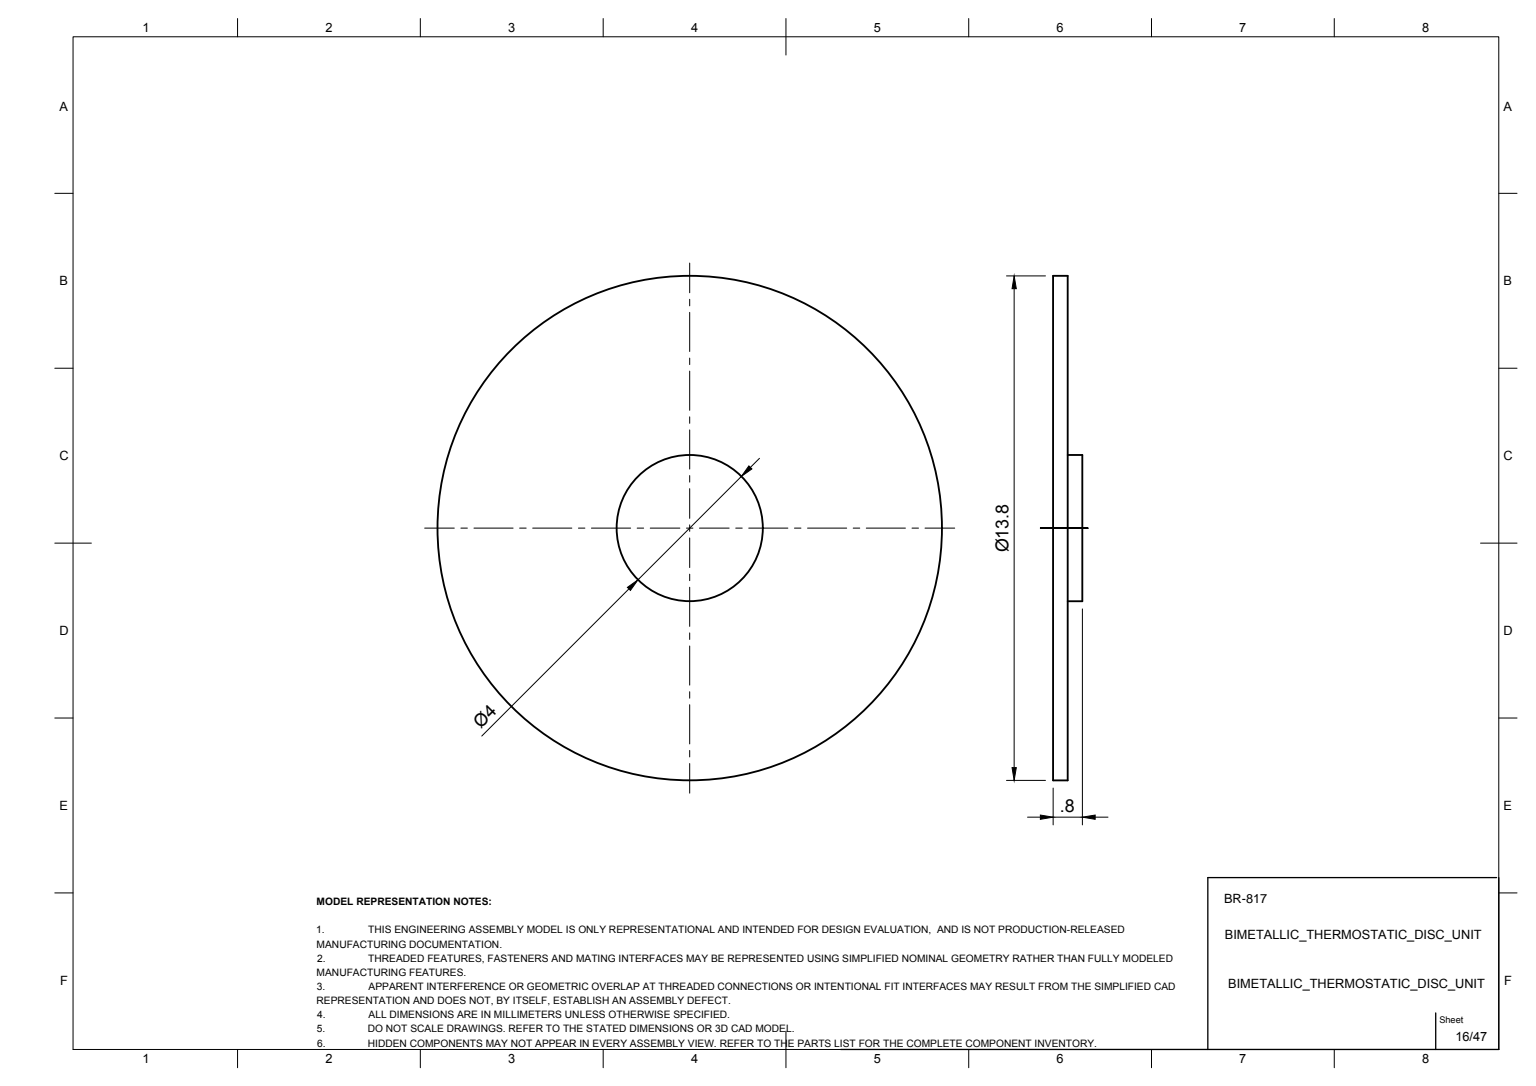
ISO-10303-21;
HEADER;
FILE_DESCRIPTION((''),'2;1');
FILE_NAME('BIMETALLIC_THERMOSTATIC_DISC_UNIT.step','2026-10-01T22:07:29-07:00',(''),(''),'','','');
FILE_SCHEMA (('AUTOMOTIVE_DESIGN { 1 0 10303 214 3 1 1 }'));
ENDSEC;
DATA;
#10=MECHANICAL_DESIGN_GEOMETRIC_PRESENTATION_REPRESENTATION('',(#550),#15484);
#480=SHAPE_REPRESENTATION_RELATIONSHIP('SRR','None',#15629,#515) ;
#515=ADVANCED_BREP_SHAPE_REPRESENTATION('',(#592),#15453) ;
#550=STYLED_ITEM('',(#15835),#592) ;
#592=MANIFOLD_SOLID_BREP('BIMETALLIC_THERMOSTATIC_DISC_UNIT',#8259) ;
#660=CYLINDRICAL_SURFACE('',#8884,0.2) ;
#661=CYLINDRICAL_SURFACE('',#8888,0.69) ;
#852=FACE_BOUND('',#2027,.T.) ;
#954=CIRCLE('',#8885,0.2) ;
#955=CIRCLE('',#8886,0.2) ;
#956=CIRCLE('',#8889,0.69) ;
#957=CIRCLE('',#8890,0.69) ;
#1480=FACE_OUTER_BOUND('',#2022,.T.) ;
#1481=FACE_OUTER_BOUND('',#2023,.T.) ;
#1482=FACE_OUTER_BOUND('',#2024,.T.) ;
#1483=FACE_OUTER_BOUND('',#2025,.T.) ;
#1484=FACE_OUTER_BOUND('',#2026,.T.) ;
#2022=EDGE_LOOP('',(#5761,#5762,#5763,#5764)) ;
#2023=EDGE_LOOP('',(#5765)) ;
#2024=EDGE_LOOP('',(#5766,#5767,#5768,#5769)) ;
#2025=EDGE_LOOP('',(#5770)) ;
#2026=EDGE_LOOP('',(#5771)) ;
#2027=EDGE_LOOP('',(#5772)) ;
#2615=LINE('',#13429,#3089) ;
#2616=LINE('',#13436,#3090) ;
#3089=VECTOR('',#10508,0.2) ;
#3090=VECTOR('',#10517,0.69) ;
#3551=VERTEX_POINT('',#13426) ;
#3552=VERTEX_POINT('',#13428) ;
#3553=VERTEX_POINT('',#13433) ;
#3554=VERTEX_POINT('',#13435) ;
#4385=EDGE_CURVE('',#3551,#3551,#954,.T.) ;
#4386=EDGE_CURVE('',#3551,#3552,#2615,.T.) ;
#4387=EDGE_CURVE('',#3552,#3552,#955,.T.) ;
#4388=EDGE_CURVE('',#3553,#3553,#956,.T.) ;
#4389=EDGE_CURVE('',#3553,#3554,#2616,.T.) ;
#4390=EDGE_CURVE('',#3554,#3554,#957,.T.) ;
#5761=ORIENTED_EDGE('',*,*,#4385,.F.) ;
#5762=ORIENTED_EDGE('',*,*,#4386,.T.) ;
#5763=ORIENTED_EDGE('',*,*,#4387,.F.) ;
#5764=ORIENTED_EDGE('',*,*,#4386,.F.) ;
#5765=ORIENTED_EDGE('',*,*,#4385,.T.) ;
#5766=ORIENTED_EDGE('',*,*,#4388,.F.) ;
#5767=ORIENTED_EDGE('',*,*,#4389,.T.) ;
#5768=ORIENTED_EDGE('',*,*,#4390,.F.) ;
#5769=ORIENTED_EDGE('',*,*,#4389,.F.) ;
#5770=ORIENTED_EDGE('',*,*,#4390,.T.) ;
#5771=ORIENTED_EDGE('',*,*,#4388,.T.) ;
#5772=ORIENTED_EDGE('',*,*,#4387,.T.) ;
#7617=PLANE('',#8887) ;
#7618=PLANE('',#8891) ;
#7619=PLANE('',#8892) ;
#7867=ADVANCED_FACE('',(#1480),#660,.T.) ;
#7868=ADVANCED_FACE('',(#1481),#7617,.T.) ;
#7869=ADVANCED_FACE('',(#1482),#661,.T.) ;
#7870=ADVANCED_FACE('',(#1483),#7618,.T.) ;
#7871=ADVANCED_FACE('',(#1484,#852),#7619,.T.) ;
#8259=CLOSED_SHELL('',(#7867,#7868,#7869,#7870,#7871)) ;
#8883=AXIS2_PLACEMENT_3D('',#13424,#10502,#10503) ;
#8884=AXIS2_PLACEMENT_3D('',#13425,#10504,#10505) ;
#8885=AXIS2_PLACEMENT_3D('',#13427,#10506,#10507) ;
#8886=AXIS2_PLACEMENT_3D('',#13430,#10509,#10510) ;
#8887=AXIS2_PLACEMENT_3D('',#13431,#10511,#10512) ;
#8888=AXIS2_PLACEMENT_3D('',#13432,#10513,#10514) ;
#8889=AXIS2_PLACEMENT_3D('',#13434,#10515,#10516) ;
#8890=AXIS2_PLACEMENT_3D('',#13437,#10518,#10519) ;
#8891=AXIS2_PLACEMENT_3D('',#13438,#10520,#10521) ;
#8892=AXIS2_PLACEMENT_3D('',#13439,#10522,#10523) ;
#10502=DIRECTION('axis',(0.,0.,1.)) ;
#10503=DIRECTION('refdir',(1.,0.,0.)) ;
#10504=DIRECTION('center_axis',(0.,0.,1.)) ;
#10505=DIRECTION('ref_axis',(1.,0.,0.)) ;
#10506=DIRECTION('center_axis',(0.,0.,1.)) ;
#10507=DIRECTION('ref_axis',(1.,0.,0.)) ;
#10508=DIRECTION('',(0.,0.,-1.)) ;
#10509=DIRECTION('center_axis',(0.,0.,-1.)) ;
#10510=DIRECTION('ref_axis',(1.,0.,0.)) ;
#10511=DIRECTION('center_axis',(0.,0.,1.)) ;
#10512=DIRECTION('ref_axis',(1.,0.,0.)) ;
#10513=DIRECTION('center_axis',(0.,0.,1.)) ;
#10514=DIRECTION('ref_axis',(1.,0.,0.)) ;
#10515=DIRECTION('center_axis',(0.,0.,1.)) ;
#10516=DIRECTION('ref_axis',(1.,0.,0.)) ;
#10517=DIRECTION('',(0.,0.,-1.)) ;
#10518=DIRECTION('center_axis',(0.,0.,-1.)) ;
#10519=DIRECTION('ref_axis',(1.,0.,0.)) ;
#10520=DIRECTION('center_axis',(0.,0.,-1.)) ;
#10521=DIRECTION('ref_axis',(-1.,0.,0.)) ;
#10522=DIRECTION('center_axis',(0.,0.,1.)) ;
#10523=DIRECTION('ref_axis',(1.,0.,0.)) ;
#13424=CARTESIAN_POINT('',(0.,0.,0.)) ;
#13425=CARTESIAN_POINT('Origin',(2.,0.8,1.11)) ;
#13426=CARTESIAN_POINT('',(1.8,0.8,1.13)) ;
#13427=CARTESIAN_POINT('Origin',(2.,0.8,1.13)) ;
#13428=CARTESIAN_POINT('',(1.8,0.8,1.09)) ;
#13429=CARTESIAN_POINT('',(1.8,0.8,1.11)) ;
#13430=CARTESIAN_POINT('Origin',(2.,0.8,1.09)) ;
#13431=CARTESIAN_POINT('Origin',(2.,0.8,1.13)) ;
#13432=CARTESIAN_POINT('Origin',(2.,0.8,1.07)) ;
#13433=CARTESIAN_POINT('',(1.31,0.8,1.09)) ;
#13434=CARTESIAN_POINT('Origin',(2.,0.8,1.09)) ;
#13435=CARTESIAN_POINT('',(1.31,0.8,1.05)) ;
#13436=CARTESIAN_POINT('',(1.31,0.8,1.07)) ;
#13437=CARTESIAN_POINT('Origin',(2.,0.8,1.05)) ;
#13438=CARTESIAN_POINT('Origin',(2.,0.8,1.05)) ;
#13439=CARTESIAN_POINT('Origin',(2.,0.8,1.09)) ;
#15410=UNCERTAINTY_MEASURE_WITH_UNIT(LENGTH_MEASURE(0.001),#15485,
'DISTANCE_ACCURACY_VALUE',
'Maximum model space distance between geometric entities at asserted c
onnectivities') ;
#15441=UNCERTAINTY_MEASURE_WITH_UNIT(LENGTH_MEASURE(0.001),#15485,
'DISTANCE_ACCURACY_VALUE',
'Maximum model space distance between geometric entities at asserted c
onnectivities') ;
#15453=(
GEOMETRIC_REPRESENTATION_CONTEXT(3)
GLOBAL_UNCERTAINTY_ASSIGNED_CONTEXT((#15410))
GLOBAL_UNIT_ASSIGNED_CONTEXT((#15485,#15487,#15488))
REPRESENTATION_CONTEXT('','3D')
) ;
#15484=(
GEOMETRIC_REPRESENTATION_CONTEXT(3)
GLOBAL_UNCERTAINTY_ASSIGNED_CONTEXT((#15441))
GLOBAL_UNIT_ASSIGNED_CONTEXT((#15485,#15487,#15488))
REPRESENTATION_CONTEXT('','3D')
) ;
#15485=(
LENGTH_UNIT()
NAMED_UNIT(*)
SI_UNIT(.CENTI.,.METRE.)
) ;
#15487=(
NAMED_UNIT(*)
PLANE_ANGLE_UNIT()
SI_UNIT($,.RADIAN.)
) ;
#15488=(
NAMED_UNIT(*)
SI_UNIT($,.STERADIAN.)
SOLID_ANGLE_UNIT()
) ;
#15500=SHAPE_DEFINITION_REPRESENTATION(#15548,#15629) ;
#15548=PRODUCT_DEFINITION_SHAPE('',$,#15672) ;
#15629=SHAPE_REPRESENTATION('',(#8883),#15453) ;
#15660=PRODUCT_DEFINITION_CONTEXT('part definition',#15788,'design') ;
#15672=PRODUCT_DEFINITION('BIMETALLIC_THERMOSTATIC_DISC_UNIT',
'BIMETALLIC_THERMOSTATIC_DISC_UNIT',#15714,#15660) ;
#15714=PRODUCT_DEFINITION_FORMATION('',$,#15801) ;
#15788=APPLICATION_CONTEXT(
'Core Data for Automotive Mechanical Design Process') ;
#15789=PRODUCT_CONTEXT('part definition',#15788,'mechanical') ;
#15801=PRODUCT('BIMETALLIC_THERMOSTATIC_DISC_UNIT',
'BIMETALLIC_THERMOSTATIC_DISC_UNIT',$,(#15789)) ;
#15835=PRESENTATION_STYLE_ASSIGNMENT((#15847)) ;
#15847=SURFACE_STYLE_USAGE(.BOTH.,#15859) ;
#15859=SURFACE_SIDE_STYLE('',(#15871)) ;
#15871=SURFACE_STYLE_FILL_AREA(#15883) ;
#15883=FILL_AREA_STYLE('Stainless Steel - Satin',(#15895)) ;
#15895=FILL_AREA_STYLE_COLOUR('Stainless Steel - Satin',#15907) ;
#15907=COLOUR_RGB('Stainless Steel - Satin', 0.40784314, 0.44705882, 0.49803922) ;
ENDSEC;
END-ISO-10303-21;
